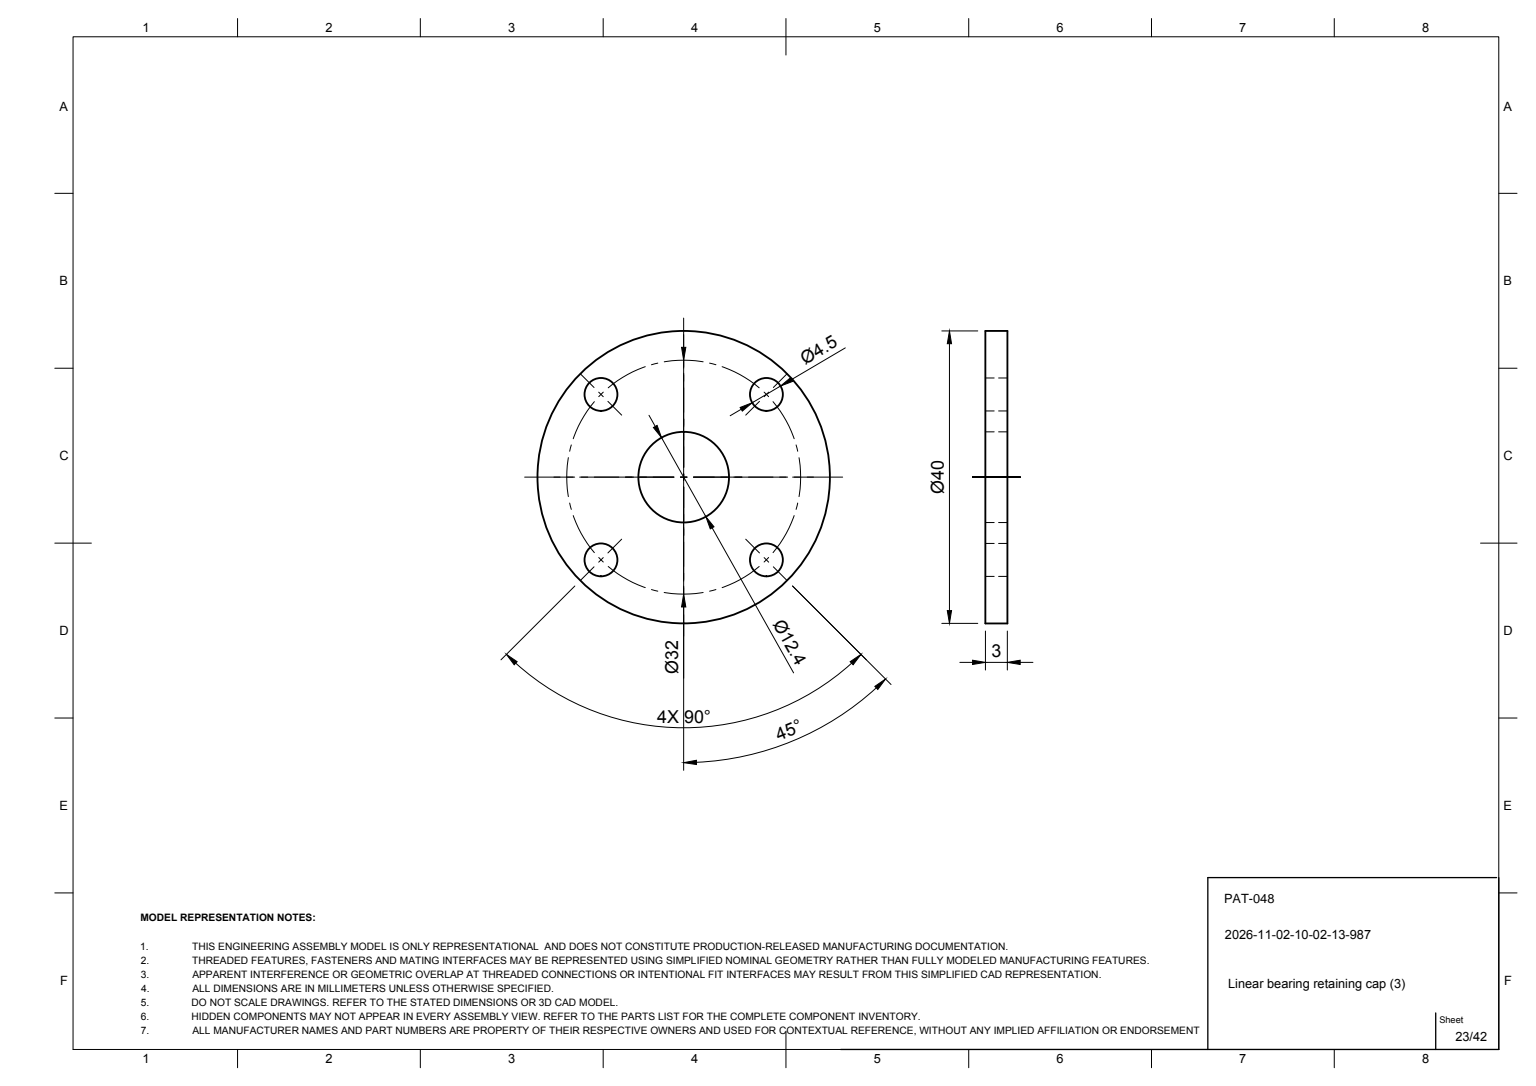
ISO-10303-21;
HEADER;
/* Generated by software containing ST-Developer
 * from STEP Tools, Inc. (www.steptools.com) 
 */

FILE_DESCRIPTION(
/* description */ ('Guided pneumatic stop gate'),
/* implementation_level */ '2;1');

FILE_NAME(
/* name */ 'Linear bearing retaining cap (3).step',
/* time_stamp */ '2026-10-27T21:43:45-07:00',
/* author */ (''),
/* organization */ (''),
/* preprocessor_version */ 'ST-DEVELOPER v20.2',
/* originating_system */ 'Autodesk Translation Framework v15.17.0.0',
/* authorisation */ '');

FILE_SCHEMA (('AUTOMOTIVE_DESIGN { 1 0 10303 214 3 1 1 }'));
ENDSEC;

DATA;
#10=MECHANICAL_DESIGN_GEOMETRIC_PRESENTATION_REPRESENTATION('',(#558),#14392);
#474=SHAPE_REPRESENTATION_RELATIONSHIP('SRR','None',#14609,#516);
#516=ADVANCED_BREP_SHAPE_REPRESENTATION('',(#599),#14371);
#558=STYLED_ITEM('',(#14891),#599);
#599=MANIFOLD_SOLID_BREP('Body1',#7899);
#767=FACE_BOUND('',#2042,.T.);
#768=FACE_BOUND('',#2043,.T.);
#769=FACE_BOUND('',#2044,.T.);
#770=FACE_BOUND('',#2045,.T.);
#771=FACE_BOUND('',#2046,.T.);
#772=FACE_BOUND('',#2048,.T.);
#773=FACE_BOUND('',#2049,.T.);
#774=FACE_BOUND('',#2050,.T.);
#775=FACE_BOUND('',#2051,.T.);
#776=FACE_BOUND('',#2052,.T.);
#1001=PLANE('',#8978);
#1002=PLANE('',#8979);
#1408=FACE_OUTER_BOUND('',#2035,.T.);
#1409=FACE_OUTER_BOUND('',#2036,.T.);
#1410=FACE_OUTER_BOUND('',#2037,.T.);
#1411=FACE_OUTER_BOUND('',#2038,.T.);
#1412=FACE_OUTER_BOUND('',#2039,.T.);
#1413=FACE_OUTER_BOUND('',#2040,.T.);
#1414=FACE_OUTER_BOUND('',#2041,.T.);
#1415=FACE_OUTER_BOUND('',#2047,.T.);
#2035=EDGE_LOOP('',(#6510,#6511,#6512,#6513));
#2036=EDGE_LOOP('',(#6514,#6515,#6516,#6517));
#2037=EDGE_LOOP('',(#6518,#6519,#6520,#6521));
#2038=EDGE_LOOP('',(#6522,#6523,#6524,#6525));
#2039=EDGE_LOOP('',(#6526,#6527,#6528,#6529));
#2040=EDGE_LOOP('',(#6530,#6531,#6532,#6533));
#2041=EDGE_LOOP('',(#6534));
#2042=EDGE_LOOP('',(#6535));
#2043=EDGE_LOOP('',(#6536));
#2044=EDGE_LOOP('',(#6537));
#2045=EDGE_LOOP('',(#6538));
#2046=EDGE_LOOP('',(#6539));
#2047=EDGE_LOOP('',(#6540));
#2048=EDGE_LOOP('',(#6541));
#2049=EDGE_LOOP('',(#6542));
#2050=EDGE_LOOP('',(#6543));
#2051=EDGE_LOOP('',(#6544));
#2052=EDGE_LOOP('',(#6545));
#2606=LINE('',#13247,#3151);
#2607=LINE('',#13253,#3152);
#2608=LINE('',#13259,#3153);
#2609=LINE('',#13265,#3154);
#2610=LINE('',#13271,#3155);
#2611=LINE('',#13277,#3156);
#3151=VECTOR('',#10865,0.225);
#3152=VECTOR('',#10872,0.225);
#3153=VECTOR('',#10879,0.225);
#3154=VECTOR('',#10886,0.225);
#3155=VECTOR('',#10893,0.62);
#3156=VECTOR('',#10900,2.);
#3611=CIRCLE('',#8961,0.225);
#3612=CIRCLE('',#8962,0.225);
#3613=CIRCLE('',#8964,0.225);
#3614=CIRCLE('',#8965,0.225);
#3615=CIRCLE('',#8967,0.225);
#3616=CIRCLE('',#8968,0.225);
#3617=CIRCLE('',#8970,0.225);
#3618=CIRCLE('',#8971,0.225);
#3619=CIRCLE('',#8973,0.62);
#3620=CIRCLE('',#8974,0.62);
#3621=CIRCLE('',#8976,2.);
#3622=CIRCLE('',#8977,2.);
#4120=VERTEX_POINT('',#13244);
#4121=VERTEX_POINT('',#13246);
#4122=VERTEX_POINT('',#13250);
#4123=VERTEX_POINT('',#13252);
#4124=VERTEX_POINT('',#13256);
#4125=VERTEX_POINT('',#13258);
#4126=VERTEX_POINT('',#13262);
#4127=VERTEX_POINT('',#13264);
#4128=VERTEX_POINT('',#13268);
#4129=VERTEX_POINT('',#13270);
#4130=VERTEX_POINT('',#13274);
#4131=VERTEX_POINT('',#13276);
#4953=EDGE_CURVE('',#4120,#4120,#3611,.T.);
#4954=EDGE_CURVE('',#4120,#4121,#2606,.T.);
#4955=EDGE_CURVE('',#4121,#4121,#3612,.T.);
#4956=EDGE_CURVE('',#4122,#4122,#3613,.T.);
#4957=EDGE_CURVE('',#4122,#4123,#2607,.T.);
#4958=EDGE_CURVE('',#4123,#4123,#3614,.T.);
#4959=EDGE_CURVE('',#4124,#4124,#3615,.T.);
#4960=EDGE_CURVE('',#4124,#4125,#2608,.T.);
#4961=EDGE_CURVE('',#4125,#4125,#3616,.T.);
#4962=EDGE_CURVE('',#4126,#4126,#3617,.T.);
#4963=EDGE_CURVE('',#4126,#4127,#2609,.T.);
#4964=EDGE_CURVE('',#4127,#4127,#3618,.T.);
#4965=EDGE_CURVE('',#4128,#4128,#3619,.T.);
#4966=EDGE_CURVE('',#4128,#4129,#2610,.T.);
#4967=EDGE_CURVE('',#4129,#4129,#3620,.T.);
#4968=EDGE_CURVE('',#4130,#4130,#3621,.T.);
#4969=EDGE_CURVE('',#4130,#4131,#2611,.T.);
#4970=EDGE_CURVE('',#4131,#4131,#3622,.T.);
#6510=ORIENTED_EDGE('',*,*,#4953,.F.);
#6511=ORIENTED_EDGE('',*,*,#4954,.T.);
#6512=ORIENTED_EDGE('',*,*,#4955,.F.);
#6513=ORIENTED_EDGE('',*,*,#4954,.F.);
#6514=ORIENTED_EDGE('',*,*,#4956,.F.);
#6515=ORIENTED_EDGE('',*,*,#4957,.T.);
#6516=ORIENTED_EDGE('',*,*,#4958,.F.);
#6517=ORIENTED_EDGE('',*,*,#4957,.F.);
#6518=ORIENTED_EDGE('',*,*,#4959,.F.);
#6519=ORIENTED_EDGE('',*,*,#4960,.T.);
#6520=ORIENTED_EDGE('',*,*,#4961,.F.);
#6521=ORIENTED_EDGE('',*,*,#4960,.F.);
#6522=ORIENTED_EDGE('',*,*,#4962,.F.);
#6523=ORIENTED_EDGE('',*,*,#4963,.T.);
#6524=ORIENTED_EDGE('',*,*,#4964,.F.);
#6525=ORIENTED_EDGE('',*,*,#4963,.F.);
#6526=ORIENTED_EDGE('',*,*,#4965,.F.);
#6527=ORIENTED_EDGE('',*,*,#4966,.T.);
#6528=ORIENTED_EDGE('',*,*,#4967,.T.);
#6529=ORIENTED_EDGE('',*,*,#4966,.F.);
#6530=ORIENTED_EDGE('',*,*,#4968,.F.);
#6531=ORIENTED_EDGE('',*,*,#4969,.T.);
#6532=ORIENTED_EDGE('',*,*,#4970,.T.);
#6533=ORIENTED_EDGE('',*,*,#4969,.F.);
#6534=ORIENTED_EDGE('',*,*,#4968,.T.);
#6535=ORIENTED_EDGE('',*,*,#4965,.T.);
#6536=ORIENTED_EDGE('',*,*,#4964,.T.);
#6537=ORIENTED_EDGE('',*,*,#4961,.T.);
#6538=ORIENTED_EDGE('',*,*,#4958,.T.);
#6539=ORIENTED_EDGE('',*,*,#4955,.T.);
#6540=ORIENTED_EDGE('',*,*,#4970,.F.);
#6541=ORIENTED_EDGE('',*,*,#4967,.F.);
#6542=ORIENTED_EDGE('',*,*,#4962,.T.);
#6543=ORIENTED_EDGE('',*,*,#4959,.T.);
#6544=ORIENTED_EDGE('',*,*,#4956,.T.);
#6545=ORIENTED_EDGE('',*,*,#4953,.T.);
#7351=CYLINDRICAL_SURFACE('',#8960,0.225);
#7352=CYLINDRICAL_SURFACE('',#8963,0.225);
#7353=CYLINDRICAL_SURFACE('',#8966,0.225);
#7354=CYLINDRICAL_SURFACE('',#8969,0.225);
#7355=CYLINDRICAL_SURFACE('',#8972,0.62);
#7356=CYLINDRICAL_SURFACE('',#8975,2.);
#7690=ADVANCED_FACE('',(#1408),#7351,.F.);
#7691=ADVANCED_FACE('',(#1409),#7352,.F.);
#7692=ADVANCED_FACE('',(#1410),#7353,.F.);
#7693=ADVANCED_FACE('',(#1411),#7354,.F.);
#7694=ADVANCED_FACE('',(#1412),#7355,.F.);
#7695=ADVANCED_FACE('',(#1413),#7356,.T.);
#7696=ADVANCED_FACE('',(#1414,#767,#768,#769,#770,#771),#1001,.T.);
#7697=ADVANCED_FACE('',(#1415,#772,#773,#774,#775,#776),#1002,.F.);
#7899=CLOSED_SHELL('',(#7690,#7691,#7692,#7693,#7694,#7695,#7696,#7697));
#8959=AXIS2_PLACEMENT_3D('',#13242,#10859,#10860);
#8960=AXIS2_PLACEMENT_3D('',#13243,#10861,#10862);
#8961=AXIS2_PLACEMENT_3D('',#13245,#10863,#10864);
#8962=AXIS2_PLACEMENT_3D('',#13248,#10866,#10867);
#8963=AXIS2_PLACEMENT_3D('',#13249,#10868,#10869);
#8964=AXIS2_PLACEMENT_3D('',#13251,#10870,#10871);
#8965=AXIS2_PLACEMENT_3D('',#13254,#10873,#10874);
#8966=AXIS2_PLACEMENT_3D('',#13255,#10875,#10876);
#8967=AXIS2_PLACEMENT_3D('',#13257,#10877,#10878);
#8968=AXIS2_PLACEMENT_3D('',#13260,#10880,#10881);
#8969=AXIS2_PLACEMENT_3D('',#13261,#10882,#10883);
#8970=AXIS2_PLACEMENT_3D('',#13263,#10884,#10885);
#8971=AXIS2_PLACEMENT_3D('',#13266,#10887,#10888);
#8972=AXIS2_PLACEMENT_3D('',#13267,#10889,#10890);
#8973=AXIS2_PLACEMENT_3D('',#13269,#10891,#10892);
#8974=AXIS2_PLACEMENT_3D('',#13272,#10894,#10895);
#8975=AXIS2_PLACEMENT_3D('',#13273,#10896,#10897);
#8976=AXIS2_PLACEMENT_3D('',#13275,#10898,#10899);
#8977=AXIS2_PLACEMENT_3D('',#13278,#10901,#10902);
#8978=AXIS2_PLACEMENT_3D('',#13279,#10903,#10904);
#8979=AXIS2_PLACEMENT_3D('',#13280,#10905,#10906);
#10859=DIRECTION('axis',(0.,0.,1.));
#10860=DIRECTION('refdir',(1.,0.,0.));
#10861=DIRECTION('center_axis',(0.,1.,0.));
#10862=DIRECTION('ref_axis',(1.,0.,0.));
#10863=DIRECTION('center_axis',(0.,1.,0.));
#10864=DIRECTION('ref_axis',(1.,0.,0.));
#10865=DIRECTION('',(0.,1.,0.));
#10866=DIRECTION('center_axis',(0.,-1.,0.));
#10867=DIRECTION('ref_axis',(1.,0.,0.));
#10868=DIRECTION('center_axis',(0.,1.,0.));
#10869=DIRECTION('ref_axis',(1.,0.,0.));
#10870=DIRECTION('center_axis',(0.,1.,0.));
#10871=DIRECTION('ref_axis',(1.,0.,0.));
#10872=DIRECTION('',(0.,1.,0.));
#10873=DIRECTION('center_axis',(0.,-1.,0.));
#10874=DIRECTION('ref_axis',(1.,0.,0.));
#10875=DIRECTION('center_axis',(0.,1.,0.));
#10876=DIRECTION('ref_axis',(1.,0.,0.));
#10877=DIRECTION('center_axis',(0.,1.,0.));
#10878=DIRECTION('ref_axis',(1.,0.,0.));
#10879=DIRECTION('',(0.,1.,0.));
#10880=DIRECTION('center_axis',(0.,-1.,0.));
#10881=DIRECTION('ref_axis',(1.,0.,0.));
#10882=DIRECTION('center_axis',(0.,1.,0.));
#10883=DIRECTION('ref_axis',(1.,0.,0.));
#10884=DIRECTION('center_axis',(0.,1.,0.));
#10885=DIRECTION('ref_axis',(1.,0.,0.));
#10886=DIRECTION('',(0.,1.,0.));
#10887=DIRECTION('center_axis',(0.,-1.,0.));
#10888=DIRECTION('ref_axis',(1.,0.,0.));
#10889=DIRECTION('center_axis',(0.,1.,0.));
#10890=DIRECTION('ref_axis',(1.,0.,0.));
#10891=DIRECTION('center_axis',(0.,-1.,0.));
#10892=DIRECTION('ref_axis',(1.,0.,0.));
#10893=DIRECTION('',(0.,-1.,0.));
#10894=DIRECTION('center_axis',(0.,-1.,0.));
#10895=DIRECTION('ref_axis',(1.,0.,0.));
#10896=DIRECTION('center_axis',(0.,1.,0.));
#10897=DIRECTION('ref_axis',(1.,0.,0.));
#10898=DIRECTION('center_axis',(0.,1.,0.));
#10899=DIRECTION('ref_axis',(1.,0.,0.));
#10900=DIRECTION('',(0.,-1.,0.));
#10901=DIRECTION('center_axis',(0.,1.,0.));
#10902=DIRECTION('ref_axis',(1.,0.,0.));
#10903=DIRECTION('center_axis',(0.,1.,0.));
#10904=DIRECTION('ref_axis',(1.,0.,0.));
#10905=DIRECTION('center_axis',(0.,1.,0.));
#10906=DIRECTION('ref_axis',(1.,0.,0.));
#13242=CARTESIAN_POINT('',(0.,0.,0.));
#13243=CARTESIAN_POINT('Origin',(3.86862915010152,8.9,3.36862915010152));
#13244=CARTESIAN_POINT('',(3.64362915010152,9.,3.36862915010152));
#13245=CARTESIAN_POINT('Origin',(3.86862915010152,9.,3.36862915010152));
#13246=CARTESIAN_POINT('',(3.64362915010152,9.3,3.36862915010152));
#13247=CARTESIAN_POINT('',(3.64362915010152,8.9,3.36862915010152));
#13248=CARTESIAN_POINT('Origin',(3.86862915010152,9.3,3.36862915010152));
#13249=CARTESIAN_POINT('Origin',(3.86862915010152,8.9,5.63137084989848));
#13250=CARTESIAN_POINT('',(3.64362915010152,9.,5.63137084989848));
#13251=CARTESIAN_POINT('Origin',(3.86862915010152,9.,5.63137084989848));
#13252=CARTESIAN_POINT('',(3.64362915010152,9.3,5.63137084989848));
#13253=CARTESIAN_POINT('',(3.64362915010152,8.9,5.63137084989848));
#13254=CARTESIAN_POINT('Origin',(3.86862915010152,9.3,5.63137084989848));
#13255=CARTESIAN_POINT('Origin',(6.13137084989848,8.9,5.63137084989848));
#13256=CARTESIAN_POINT('',(5.90637084989848,9.,5.63137084989848));
#13257=CARTESIAN_POINT('Origin',(6.13137084989848,9.,5.63137084989848));
#13258=CARTESIAN_POINT('',(5.90637084989848,9.3,5.63137084989848));
#13259=CARTESIAN_POINT('',(5.90637084989848,8.9,5.63137084989848));
#13260=CARTESIAN_POINT('Origin',(6.13137084989848,9.3,5.63137084989848));
#13261=CARTESIAN_POINT('Origin',(6.13137084989848,8.9,3.36862915010152));
#13262=CARTESIAN_POINT('',(5.90637084989848,9.,3.36862915010152));
#13263=CARTESIAN_POINT('Origin',(6.13137084989848,9.,3.36862915010152));
#13264=CARTESIAN_POINT('',(5.90637084989848,9.3,3.36862915010152));
#13265=CARTESIAN_POINT('',(5.90637084989848,8.9,3.36862915010152));
#13266=CARTESIAN_POINT('Origin',(6.13137084989848,9.3,3.36862915010152));
#13267=CARTESIAN_POINT('Origin',(5.,9.,4.5));
#13268=CARTESIAN_POINT('',(4.38,9.3,4.5));
#13269=CARTESIAN_POINT('Origin',(5.,9.3,4.5));
#13270=CARTESIAN_POINT('',(4.38,9.,4.5));
#13271=CARTESIAN_POINT('',(4.38,9.,4.5));
#13272=CARTESIAN_POINT('Origin',(5.,9.,4.5));
#13273=CARTESIAN_POINT('Origin',(5.,9.,4.5));
#13274=CARTESIAN_POINT('',(3.,9.3,4.5));
#13275=CARTESIAN_POINT('Origin',(5.,9.3,4.5));
#13276=CARTESIAN_POINT('',(3.,9.,4.5));
#13277=CARTESIAN_POINT('',(3.,9.,4.5));
#13278=CARTESIAN_POINT('Origin',(5.,9.,4.5));
#13279=CARTESIAN_POINT('Origin',(5.,9.3,4.5));
#13280=CARTESIAN_POINT('Origin',(5.,9.,4.5));
#14323=UNCERTAINTY_MEASURE_WITH_UNIT(LENGTH_MEASURE(0.001),#14393,
'DISTANCE_ACCURACY_VALUE',
'Maximum model space distance between geometric entities at asserted c
onnectivities');
#14344=UNCERTAINTY_MEASURE_WITH_UNIT(LENGTH_MEASURE(0.001),#14393,
'DISTANCE_ACCURACY_VALUE',
'Maximum model space distance between geometric entities at asserted c
onnectivities');
#14371=(
GEOMETRIC_REPRESENTATION_CONTEXT(3)
GLOBAL_UNCERTAINTY_ASSIGNED_CONTEXT((#14323))
GLOBAL_UNIT_ASSIGNED_CONTEXT((#14393,#14395,#14396))
REPRESENTATION_CONTEXT('','3D')
);
#14392=(
GEOMETRIC_REPRESENTATION_CONTEXT(3)
GLOBAL_UNCERTAINTY_ASSIGNED_CONTEXT((#14344))
GLOBAL_UNIT_ASSIGNED_CONTEXT((#14393,#14395,#14396))
REPRESENTATION_CONTEXT('','3D')
);
#14393=(
LENGTH_UNIT()
NAMED_UNIT(*)
SI_UNIT(.CENTI.,.METRE.)
);
#14395=(
NAMED_UNIT(*)
PLANE_ANGLE_UNIT()
SI_UNIT($,.RADIAN.)
);
#14396=(
NAMED_UNIT(*)
SI_UNIT($,.STERADIAN.)
SOLID_ANGLE_UNIT()
);
#14423=SHAPE_DEFINITION_REPRESENTATION(#14472,#14609);
#14472=PRODUCT_DEFINITION_SHAPE('',$,#14657);
#14609=SHAPE_REPRESENTATION('',(#8959),#14371);
#14630=PRODUCT_DEFINITION_CONTEXT('part definition',#14773,'design');
#14657=PRODUCT_DEFINITION('Linear bearing retaining cap (3)',
'Linear bearing retaining cap (3)',#14704,#14630);
#14704=PRODUCT_DEFINITION_FORMATION('',$,#14801);
#14773=APPLICATION_CONTEXT(
'Core Data for Automotive Mechanical Design Process');
#14774=PRODUCT_CONTEXT('part definition',#14773,'mechanical');
#14801=PRODUCT('Linear bearing retaining cap (3)',
'Linear bearing retaining cap (3)','Linear bearing retaining cap (3)',(#14774));
#14885=COLOUR_RGB('Grey',0.48,0.52,0.57);
#14886=FILL_AREA_STYLE_COLOUR('',#14885);
#14887=FILL_AREA_STYLE('',(#14886));
#14888=SURFACE_STYLE_FILL_AREA(#14887);
#14889=SURFACE_SIDE_STYLE('',(#14888));
#14890=SURFACE_STYLE_USAGE(.BOTH.,#14889);
#14891=PRESENTATION_STYLE_ASSIGNMENT((#14890));
ENDSEC;
END-ISO-10303-21;
